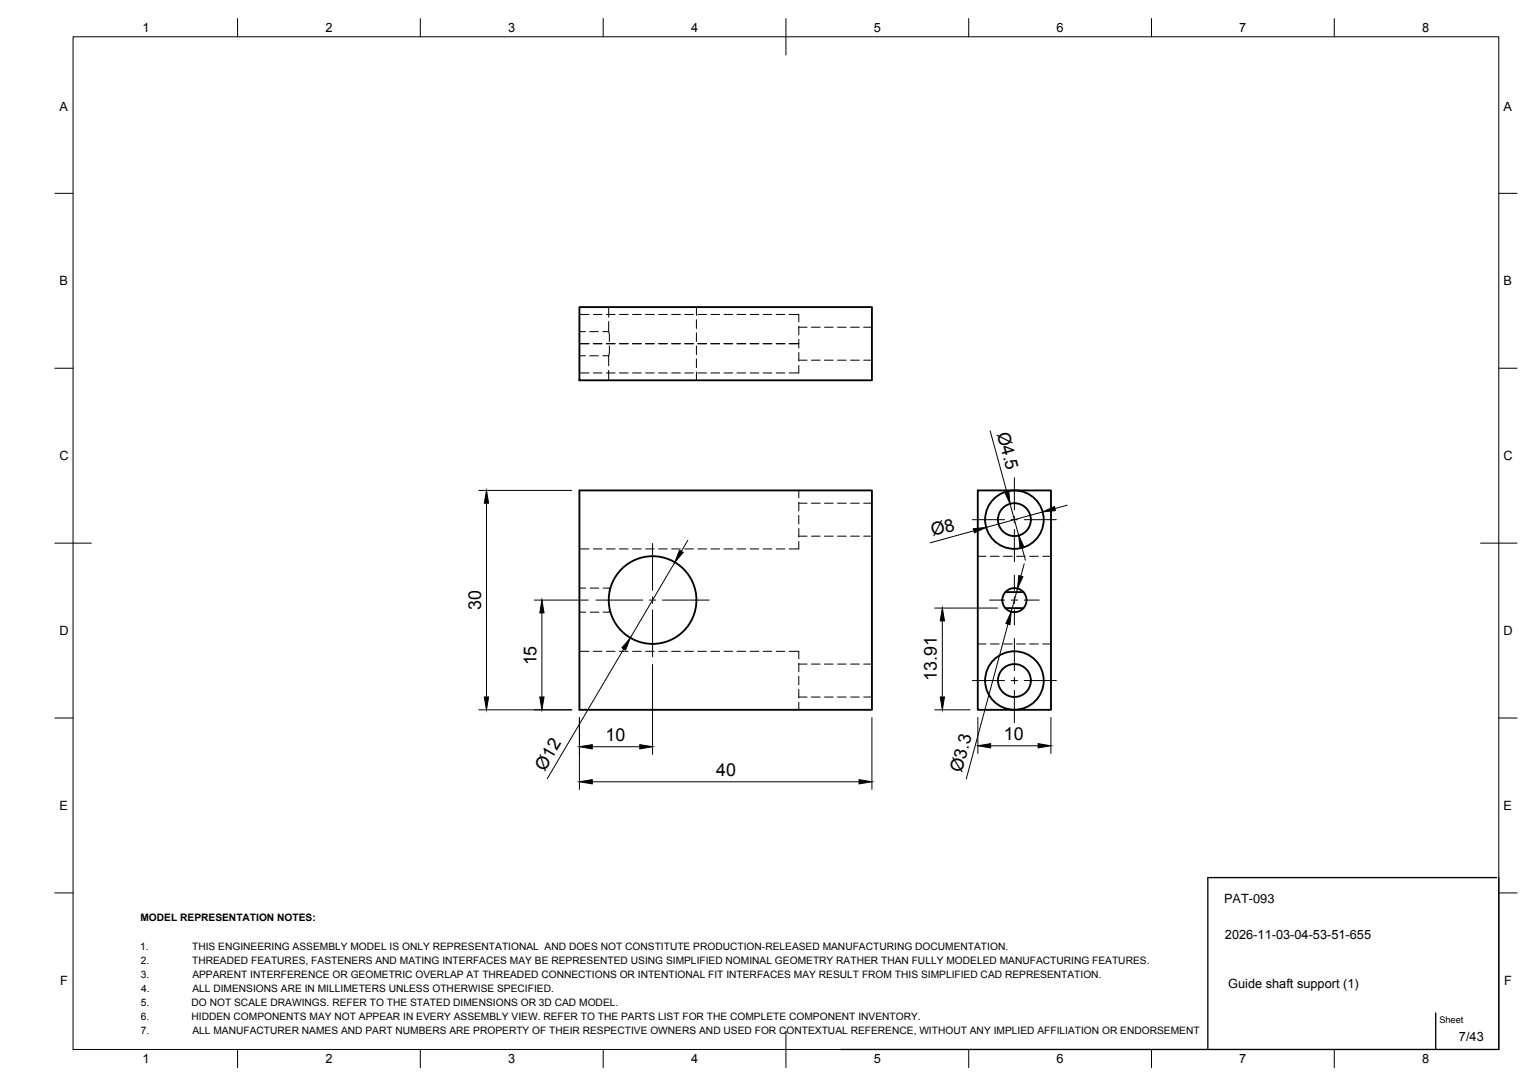
ISO-10303-21;
HEADER;
/* Generated by software containing ST-Developer
 * from STEP Tools, Inc. (www.steptools.com) 
 */

FILE_DESCRIPTION(
/* description */ ('Self-centering screw clamp'),
/* implementation_level */ '2;1');

FILE_NAME(
/* name */ 'Guide shaft support (1).step',
/* time_stamp */ '2026-10-28T03:25:31-07:00',
/* author */ (''),
/* organization */ (''),
/* preprocessor_version */ 'ST-DEVELOPER v20.2',
/* originating_system */ 'Autodesk Translation Framework v15.17.0.0',
/* authorisation */ '');

FILE_SCHEMA (('AUTOMOTIVE_DESIGN { 1 0 10303 214 3 1 1 }'));
ENDSEC;

DATA;
#10=MECHANICAL_DESIGN_GEOMETRIC_PRESENTATION_REPRESENTATION('',(#628),#16799);
#502=B_SPLINE_CURVE_WITH_KNOTS('',3,(#13973,#13974,#13975,#13976,#13977,
#13978),.UNSPECIFIED.,.F.,.F.,(4,2,4),(0.635430324955931,0.687528937234027,
0.750024497760672),.UNSPECIFIED.);
#503=B_SPLINE_CURVE_WITH_KNOTS('',3,(#13982,#13983,#13984,#13985,#13986,
#13987),.UNSPECIFIED.,.F.,.F.,(4,2,4),(0.250008165920224,0.312503726446869,
0.364602338724963),.UNSPECIFIED.);
#504=B_SPLINE_CURVE_WITH_KNOTS('',3,(#13988,#13989,#13990,#13991,#13992,
#13993),.UNSPECIFIED.,.F.,.F.,(4,2,4),(0.135413993115483,0.187512605393579,
0.250008165920224),.UNSPECIFIED.);
#505=B_SPLINE_CURVE_WITH_KNOTS('',3,(#13994,#13995,#13996,#13997,#13998,
#13999),.UNSPECIFIED.,.F.,.F.,(4,2,4),(0.750024497760672,0.812520058287317,
0.864618670565414),.UNSPECIFIED.);
#546=SHAPE_REPRESENTATION_RELATIONSHIP('SRR','None',#17019,#587);
#587=ADVANCED_BREP_SHAPE_REPRESENTATION('',(#676),#16757);
#628=STYLED_ITEM('',(#17326),#676);
#676=MANIFOLD_SOLID_BREP('Body1',#9079);
#749=FACE_BOUND('',#1863,.T.);
#750=FACE_BOUND('',#1866,.T.);
#751=FACE_BOUND('',#1868,.T.);
#752=FACE_BOUND('',#1874,.T.);
#753=FACE_BOUND('',#1877,.T.);
#754=FACE_BOUND('',#1879,.T.);
#755=FACE_BOUND('',#1880,.T.);
#1042=PLANE('',#9679);
#1043=PLANE('',#9684);
#1044=PLANE('',#9688);
#1045=PLANE('',#9693);
#1046=PLANE('',#9695);
#1047=PLANE('',#9703);
#1048=PLANE('',#9704);
#1049=PLANE('',#9705);
#1050=PLANE('',#9706);
#1051=PLANE('',#9707);
#1321=FACE_OUTER_BOUND('',#1856,.T.);
#1322=FACE_OUTER_BOUND('',#1857,.T.);
#1323=FACE_OUTER_BOUND('',#1858,.T.);
#1324=FACE_OUTER_BOUND('',#1859,.T.);
#1325=FACE_OUTER_BOUND('',#1860,.T.);
#1326=FACE_OUTER_BOUND('',#1861,.T.);
#1327=FACE_OUTER_BOUND('',#1862,.T.);
#1328=FACE_OUTER_BOUND('',#1864,.T.);
#1329=FACE_OUTER_BOUND('',#1865,.T.);
#1330=FACE_OUTER_BOUND('',#1867,.T.);
#1331=FACE_OUTER_BOUND('',#1869,.T.);
#1332=FACE_OUTER_BOUND('',#1870,.T.);
#1333=FACE_OUTER_BOUND('',#1871,.T.);
#1334=FACE_OUTER_BOUND('',#1872,.T.);
#1335=FACE_OUTER_BOUND('',#1873,.T.);
#1336=FACE_OUTER_BOUND('',#1875,.T.);
#1337=FACE_OUTER_BOUND('',#1876,.T.);
#1338=FACE_OUTER_BOUND('',#1878,.T.);
#1856=EDGE_LOOP('',(#6343,#6344,#6345,#6346));
#1857=EDGE_LOOP('',(#6347,#6348,#6349,#6350));
#1858=EDGE_LOOP('',(#6351,#6352));
#1859=EDGE_LOOP('',(#6353,#6354,#6355,#6356,#6357,#6358,#6359,#6360,#6361));
#1860=EDGE_LOOP('',(#6362,#6363));
#1861=EDGE_LOOP('',(#6364,#6365,#6366,#6367));
#1862=EDGE_LOOP('',(#6368,#6369));
#1863=EDGE_LOOP('',(#6370));
#1864=EDGE_LOOP('',(#6371,#6372,#6373,#6374));
#1865=EDGE_LOOP('',(#6375,#6376));
#1866=EDGE_LOOP('',(#6377));
#1867=EDGE_LOOP('',(#6378,#6379,#6380,#6381,#6382,#6383,#6384,#6385,#6386,
#6387));
#1868=EDGE_LOOP('',(#6388));
#1869=EDGE_LOOP('',(#6389,#6390,#6391,#6392));
#1870=EDGE_LOOP('',(#6393,#6394,#6395,#6396));
#1871=EDGE_LOOP('',(#6397,#6398,#6399,#6400,#6401,#6402,#6403,#6404,#6405,
#6406,#6407,#6408));
#1872=EDGE_LOOP('',(#6409,#6410,#6411,#6412,#6413,#6414,#6415));
#1873=EDGE_LOOP('',(#6416,#6417,#6418,#6419));
#1874=EDGE_LOOP('',(#6420));
#1875=EDGE_LOOP('',(#6421,#6422,#6423,#6424,#6425,#6426,#6427));
#1876=EDGE_LOOP('',(#6428,#6429,#6430,#6431));
#1877=EDGE_LOOP('',(#6432));
#1878=EDGE_LOOP('',(#6433,#6434,#6435,#6436));
#1879=EDGE_LOOP('',(#6437));
#1880=EDGE_LOOP('',(#6438));
#2652=LINE('',#13950,#3225);
#2653=LINE('',#13954,#3226);
#2654=LINE('',#13959,#3227);
#2655=LINE('',#13963,#3228);
#2656=LINE('',#13968,#3229);
#2657=LINE('',#14001,#3230);
#2658=LINE('',#14004,#3231);
#2659=LINE('',#14007,#3232);
#2660=LINE('',#14014,#3233);
#2661=LINE('',#14022,#3234);
#2662=LINE('',#14023,#3235);
#2663=LINE('',#14025,#3236);
#2664=LINE('',#14027,#3237);
#2665=LINE('',#14028,#3238);
#2666=LINE('',#14029,#3239);
#2667=LINE('',#14033,#3240);
#2668=LINE('',#14037,#3241);
#2669=LINE('',#14041,#3242);
#2670=LINE('',#14043,#3243);
#2671=LINE('',#14048,#3244);
#2672=LINE('',#14049,#3245);
#2673=LINE('',#14050,#3246);
#2674=LINE('',#14053,#3247);
#2675=LINE('',#14054,#3248);
#2676=LINE('',#14057,#3249);
#2677=LINE('',#14058,#3250);
#2678=LINE('',#14060,#3251);
#3225=VECTOR('',#11021,0.4);
#3226=VECTOR('',#11024,1.);
#3227=VECTOR('',#11029,0.4);
#3228=VECTOR('',#11032,1.);
#3229=VECTOR('',#11037,1.);
#3230=VECTOR('',#11044,0.164999999999999);
#3231=VECTOR('',#11049,1.);
#3232=VECTOR('',#11054,1.);
#3233=VECTOR('',#11065,1.);
#3234=VECTOR('',#11074,1.);
#3235=VECTOR('',#11075,1.);
#3236=VECTOR('',#11076,1.);
#3237=VECTOR('',#11077,1.);
#3238=VECTOR('',#11078,1.);
#3239=VECTOR('',#11079,1.);
#3240=VECTOR('',#11084,0.225);
#3241=VECTOR('',#11089,0.225);
#3242=VECTOR('',#11094,0.6);
#3243=VECTOR('',#11095,0.6);
#3244=VECTOR('',#11100,1.);
#3245=VECTOR('',#11101,1.);
#3246=VECTOR('',#11102,1.);
#3247=VECTOR('',#11105,1.);
#3248=VECTOR('',#11106,1.);
#3249=VECTOR('',#11109,1.);
#3250=VECTOR('',#11110,1.);
#3251=VECTOR('',#11113,1.);
#3764=CIRCLE('',#9674,0.4);
#3765=CIRCLE('',#9675,0.4);
#3766=CIRCLE('',#9677,0.4);
#3767=CIRCLE('',#9678,0.4);
#3768=CIRCLE('',#9680,0.164999999999999);
#3769=CIRCLE('',#9682,0.164999999999999);
#3770=CIRCLE('',#9683,0.164999999999999);
#3771=CIRCLE('',#9686,0.4);
#3772=CIRCLE('',#9687,0.4);
#3773=CIRCLE('',#9689,0.225);
#3774=CIRCLE('',#9691,0.4);
#3775=CIRCLE('',#9692,0.4);
#3776=CIRCLE('',#9694,0.225);
#3777=CIRCLE('',#9697,0.225);
#3778=CIRCLE('',#9699,0.225);
#3779=CIRCLE('',#9701,0.6);
#3780=CIRCLE('',#9702,0.6);
#4310=VERTEX_POINT('',#13948);
#4311=VERTEX_POINT('',#13949);
#4312=VERTEX_POINT('',#13951);
#4313=VERTEX_POINT('',#13953);
#4314=VERTEX_POINT('',#13957);
#4315=VERTEX_POINT('',#13958);
#4316=VERTEX_POINT('',#13960);
#4317=VERTEX_POINT('',#13962);
#4318=VERTEX_POINT('',#13966);
#4319=VERTEX_POINT('',#13967);
#4320=VERTEX_POINT('',#13971);
#4321=VERTEX_POINT('',#13972);
#4322=VERTEX_POINT('',#13979);
#4323=VERTEX_POINT('',#13981);
#4324=VERTEX_POINT('',#14000);
#4325=VERTEX_POINT('',#14010);
#4326=VERTEX_POINT('',#14017);
#4327=VERTEX_POINT('',#14020);
#4328=VERTEX_POINT('',#14021);
#4329=VERTEX_POINT('',#14024);
#4330=VERTEX_POINT('',#14026);
#4331=VERTEX_POINT('',#14031);
#4332=VERTEX_POINT('',#14035);
#4333=VERTEX_POINT('',#14039);
#4334=VERTEX_POINT('',#14042);
#4335=VERTEX_POINT('',#14046);
#4336=VERTEX_POINT('',#14047);
#4337=VERTEX_POINT('',#14052);
#4338=VERTEX_POINT('',#14056);
#5096=EDGE_CURVE('',#4310,#4311,#2652,.T.);
#5097=EDGE_CURVE('',#4312,#4310,#3764,.T.);
#5098=EDGE_CURVE('',#4312,#4313,#2653,.T.);
#5099=EDGE_CURVE('',#4311,#4313,#3765,.T.);
#5100=EDGE_CURVE('',#4314,#4315,#2654,.T.);
#5101=EDGE_CURVE('',#4316,#4314,#3766,.T.);
#5102=EDGE_CURVE('',#4316,#4317,#2655,.T.);
#5103=EDGE_CURVE('',#4315,#4317,#3767,.T.);
#5104=EDGE_CURVE('',#4318,#4319,#2656,.T.);
#5105=EDGE_CURVE('',#4318,#4319,#3768,.T.);
#5106=EDGE_CURVE('',#4320,#4321,#502,.T.);
#5107=EDGE_CURVE('',#4322,#4320,#3769,.T.);
#5108=EDGE_CURVE('',#4323,#4322,#503,.T.);
#5109=EDGE_CURVE('',#4319,#4323,#504,.T.);
#5110=EDGE_CURVE('',#4321,#4318,#505,.T.);
#5111=EDGE_CURVE('',#4321,#4324,#2657,.T.);
#5112=EDGE_CURVE('',#4324,#4324,#3770,.T.);
#5113=EDGE_CURVE('',#4322,#4320,#2658,.T.);
#5114=EDGE_CURVE('',#4317,#4315,#3771,.T.);
#5115=EDGE_CURVE('',#4316,#4317,#2659,.T.);
#5116=EDGE_CURVE('',#4314,#4316,#3772,.T.);
#5117=EDGE_CURVE('',#4325,#4325,#3773,.T.);
#5118=EDGE_CURVE('',#4313,#4311,#3774,.T.);
#5119=EDGE_CURVE('',#4312,#4313,#2660,.T.);
#5120=EDGE_CURVE('',#4310,#4312,#3775,.T.);
#5121=EDGE_CURVE('',#4326,#4326,#3776,.T.);
#5122=EDGE_CURVE('',#4327,#4328,#2661,.T.);
#5123=EDGE_CURVE('',#4328,#4317,#2662,.T.);
#5124=EDGE_CURVE('',#4317,#4329,#2663,.T.);
#5125=EDGE_CURVE('',#4329,#4330,#2664,.T.);
#5126=EDGE_CURVE('',#4330,#4313,#2665,.T.);
#5127=EDGE_CURVE('',#4313,#4327,#2666,.T.);
#5128=EDGE_CURVE('',#4331,#4331,#3777,.T.);
#5129=EDGE_CURVE('',#4331,#4325,#2667,.T.);
#5130=EDGE_CURVE('',#4332,#4332,#3778,.T.);
#5131=EDGE_CURVE('',#4332,#4326,#2668,.T.);
#5132=EDGE_CURVE('',#4333,#4333,#3779,.T.);
#5133=EDGE_CURVE('',#4333,#4321,#2669,.T.);
#5134=EDGE_CURVE('',#4323,#4334,#2670,.T.);
#5135=EDGE_CURVE('',#4334,#4334,#3780,.T.);
#5136=EDGE_CURVE('',#4335,#4336,#2671,.T.);
#5137=EDGE_CURVE('',#4336,#4327,#2672,.T.);
#5138=EDGE_CURVE('',#4335,#4330,#2673,.T.);
#5139=EDGE_CURVE('',#4337,#4335,#2674,.T.);
#5140=EDGE_CURVE('',#4337,#4329,#2675,.T.);
#5141=EDGE_CURVE('',#4338,#4337,#2676,.T.);
#5142=EDGE_CURVE('',#4338,#4328,#2677,.T.);
#5143=EDGE_CURVE('',#4336,#4338,#2678,.T.);
#6343=ORIENTED_EDGE('',*,*,#5096,.F.);
#6344=ORIENTED_EDGE('',*,*,#5097,.F.);
#6345=ORIENTED_EDGE('',*,*,#5098,.T.);
#6346=ORIENTED_EDGE('',*,*,#5099,.F.);
#6347=ORIENTED_EDGE('',*,*,#5100,.F.);
#6348=ORIENTED_EDGE('',*,*,#5101,.F.);
#6349=ORIENTED_EDGE('',*,*,#5102,.T.);
#6350=ORIENTED_EDGE('',*,*,#5103,.F.);
#6351=ORIENTED_EDGE('',*,*,#5104,.F.);
#6352=ORIENTED_EDGE('',*,*,#5105,.T.);
#6353=ORIENTED_EDGE('',*,*,#5106,.F.);
#6354=ORIENTED_EDGE('',*,*,#5107,.F.);
#6355=ORIENTED_EDGE('',*,*,#5108,.F.);
#6356=ORIENTED_EDGE('',*,*,#5109,.F.);
#6357=ORIENTED_EDGE('',*,*,#5105,.F.);
#6358=ORIENTED_EDGE('',*,*,#5110,.F.);
#6359=ORIENTED_EDGE('',*,*,#5111,.T.);
#6360=ORIENTED_EDGE('',*,*,#5112,.F.);
#6361=ORIENTED_EDGE('',*,*,#5111,.F.);
#6362=ORIENTED_EDGE('',*,*,#5113,.F.);
#6363=ORIENTED_EDGE('',*,*,#5107,.T.);
#6364=ORIENTED_EDGE('',*,*,#5100,.T.);
#6365=ORIENTED_EDGE('',*,*,#5114,.F.);
#6366=ORIENTED_EDGE('',*,*,#5115,.F.);
#6367=ORIENTED_EDGE('',*,*,#5116,.F.);
#6368=ORIENTED_EDGE('',*,*,#5101,.T.);
#6369=ORIENTED_EDGE('',*,*,#5116,.T.);
#6370=ORIENTED_EDGE('',*,*,#5117,.F.);
#6371=ORIENTED_EDGE('',*,*,#5096,.T.);
#6372=ORIENTED_EDGE('',*,*,#5118,.F.);
#6373=ORIENTED_EDGE('',*,*,#5119,.F.);
#6374=ORIENTED_EDGE('',*,*,#5120,.F.);
#6375=ORIENTED_EDGE('',*,*,#5097,.T.);
#6376=ORIENTED_EDGE('',*,*,#5120,.T.);
#6377=ORIENTED_EDGE('',*,*,#5121,.F.);
#6378=ORIENTED_EDGE('',*,*,#5122,.T.);
#6379=ORIENTED_EDGE('',*,*,#5123,.T.);
#6380=ORIENTED_EDGE('',*,*,#5114,.T.);
#6381=ORIENTED_EDGE('',*,*,#5103,.T.);
#6382=ORIENTED_EDGE('',*,*,#5124,.T.);
#6383=ORIENTED_EDGE('',*,*,#5125,.T.);
#6384=ORIENTED_EDGE('',*,*,#5126,.T.);
#6385=ORIENTED_EDGE('',*,*,#5118,.T.);
#6386=ORIENTED_EDGE('',*,*,#5099,.T.);
#6387=ORIENTED_EDGE('',*,*,#5127,.T.);
#6388=ORIENTED_EDGE('',*,*,#5112,.T.);
#6389=ORIENTED_EDGE('',*,*,#5128,.F.);
#6390=ORIENTED_EDGE('',*,*,#5129,.T.);
#6391=ORIENTED_EDGE('',*,*,#5117,.T.);
#6392=ORIENTED_EDGE('',*,*,#5129,.F.);
#6393=ORIENTED_EDGE('',*,*,#5130,.F.);
#6394=ORIENTED_EDGE('',*,*,#5131,.T.);
#6395=ORIENTED_EDGE('',*,*,#5121,.T.);
#6396=ORIENTED_EDGE('',*,*,#5131,.F.);
#6397=ORIENTED_EDGE('',*,*,#5132,.F.);
#6398=ORIENTED_EDGE('',*,*,#5133,.T.);
#6399=ORIENTED_EDGE('',*,*,#5110,.T.);
#6400=ORIENTED_EDGE('',*,*,#5104,.T.);
#6401=ORIENTED_EDGE('',*,*,#5109,.T.);
#6402=ORIENTED_EDGE('',*,*,#5134,.T.);
#6403=ORIENTED_EDGE('',*,*,#5135,.F.);
#6404=ORIENTED_EDGE('',*,*,#5134,.F.);
#6405=ORIENTED_EDGE('',*,*,#5108,.T.);
#6406=ORIENTED_EDGE('',*,*,#5113,.T.);
#6407=ORIENTED_EDGE('',*,*,#5106,.T.);
#6408=ORIENTED_EDGE('',*,*,#5133,.F.);
#6409=ORIENTED_EDGE('',*,*,#5136,.T.);
#6410=ORIENTED_EDGE('',*,*,#5137,.T.);
#6411=ORIENTED_EDGE('',*,*,#5127,.F.);
#6412=ORIENTED_EDGE('',*,*,#5098,.F.);
#6413=ORIENTED_EDGE('',*,*,#5119,.T.);
#6414=ORIENTED_EDGE('',*,*,#5126,.F.);
#6415=ORIENTED_EDGE('',*,*,#5138,.F.);
#6416=ORIENTED_EDGE('',*,*,#5139,.T.);
#6417=ORIENTED_EDGE('',*,*,#5138,.T.);
#6418=ORIENTED_EDGE('',*,*,#5125,.F.);
#6419=ORIENTED_EDGE('',*,*,#5140,.F.);
#6420=ORIENTED_EDGE('',*,*,#5135,.T.);
#6421=ORIENTED_EDGE('',*,*,#5141,.T.);
#6422=ORIENTED_EDGE('',*,*,#5140,.T.);
#6423=ORIENTED_EDGE('',*,*,#5124,.F.);
#6424=ORIENTED_EDGE('',*,*,#5102,.F.);
#6425=ORIENTED_EDGE('',*,*,#5115,.T.);
#6426=ORIENTED_EDGE('',*,*,#5123,.F.);
#6427=ORIENTED_EDGE('',*,*,#5142,.F.);
#6428=ORIENTED_EDGE('',*,*,#5143,.T.);
#6429=ORIENTED_EDGE('',*,*,#5142,.T.);
#6430=ORIENTED_EDGE('',*,*,#5122,.F.);
#6431=ORIENTED_EDGE('',*,*,#5137,.F.);
#6432=ORIENTED_EDGE('',*,*,#5132,.T.);
#6433=ORIENTED_EDGE('',*,*,#5143,.F.);
#6434=ORIENTED_EDGE('',*,*,#5136,.F.);
#6435=ORIENTED_EDGE('',*,*,#5139,.F.);
#6436=ORIENTED_EDGE('',*,*,#5141,.F.);
#6437=ORIENTED_EDGE('',*,*,#5128,.T.);
#6438=ORIENTED_EDGE('',*,*,#5130,.T.);
#8377=CYLINDRICAL_SURFACE('',#9673,0.4);
#8378=CYLINDRICAL_SURFACE('',#9676,0.4);
#8379=CYLINDRICAL_SURFACE('',#9681,0.164999999999999);
#8380=CYLINDRICAL_SURFACE('',#9685,0.4);
#8381=CYLINDRICAL_SURFACE('',#9690,0.4);
#8382=CYLINDRICAL_SURFACE('',#9696,0.225);
#8383=CYLINDRICAL_SURFACE('',#9698,0.225);
#8384=CYLINDRICAL_SURFACE('',#9700,0.6);
#8619=ADVANCED_FACE('',(#1321),#8377,.F.);
#8620=ADVANCED_FACE('',(#1322),#8378,.F.);
#8621=ADVANCED_FACE('',(#1323),#1042,.T.);
#8622=ADVANCED_FACE('',(#1324),#8379,.F.);
#8623=ADVANCED_FACE('',(#1325),#1043,.T.);
#8624=ADVANCED_FACE('',(#1326),#8380,.F.);
#8625=ADVANCED_FACE('',(#1327,#749),#1044,.T.);
#8626=ADVANCED_FACE('',(#1328),#8381,.F.);
#8627=ADVANCED_FACE('',(#1329,#750),#1045,.T.);
#8628=ADVANCED_FACE('',(#1330,#751),#1046,.T.);
#8629=ADVANCED_FACE('',(#1331),#8382,.F.);
#8630=ADVANCED_FACE('',(#1332),#8383,.F.);
#8631=ADVANCED_FACE('',(#1333),#8384,.F.);
#8632=ADVANCED_FACE('',(#1334),#1047,.T.);
#8633=ADVANCED_FACE('',(#1335,#752),#1048,.T.);
#8634=ADVANCED_FACE('',(#1336),#1049,.T.);
#8635=ADVANCED_FACE('',(#1337,#753),#1050,.T.);
#8636=ADVANCED_FACE('',(#1338,#754,#755),#1051,.F.);
#9079=CLOSED_SHELL('',(#8619,#8620,#8621,#8622,#8623,#8624,#8625,#8626,
#8627,#8628,#8629,#8630,#8631,#8632,#8633,#8634,#8635,#8636));
#9672=AXIS2_PLACEMENT_3D('',#13946,#11017,#11018);
#9673=AXIS2_PLACEMENT_3D('',#13947,#11019,#11020);
#9674=AXIS2_PLACEMENT_3D('',#13952,#11022,#11023);
#9675=AXIS2_PLACEMENT_3D('',#13955,#11025,#11026);
#9676=AXIS2_PLACEMENT_3D('',#13956,#11027,#11028);
#9677=AXIS2_PLACEMENT_3D('',#13961,#11030,#11031);
#9678=AXIS2_PLACEMENT_3D('',#13964,#11033,#11034);
#9679=AXIS2_PLACEMENT_3D('',#13965,#11035,#11036);
#9680=AXIS2_PLACEMENT_3D('',#13969,#11038,#11039);
#9681=AXIS2_PLACEMENT_3D('',#13970,#11040,#11041);
#9682=AXIS2_PLACEMENT_3D('',#13980,#11042,#11043);
#9683=AXIS2_PLACEMENT_3D('',#14002,#11045,#11046);
#9684=AXIS2_PLACEMENT_3D('',#14003,#11047,#11048);
#9685=AXIS2_PLACEMENT_3D('',#14005,#11050,#11051);
#9686=AXIS2_PLACEMENT_3D('',#14006,#11052,#11053);
#9687=AXIS2_PLACEMENT_3D('',#14008,#11055,#11056);
#9688=AXIS2_PLACEMENT_3D('',#14009,#11057,#11058);
#9689=AXIS2_PLACEMENT_3D('',#14011,#11059,#11060);
#9690=AXIS2_PLACEMENT_3D('',#14012,#11061,#11062);
#9691=AXIS2_PLACEMENT_3D('',#14013,#11063,#11064);
#9692=AXIS2_PLACEMENT_3D('',#14015,#11066,#11067);
#9693=AXIS2_PLACEMENT_3D('',#14016,#11068,#11069);
#9694=AXIS2_PLACEMENT_3D('',#14018,#11070,#11071);
#9695=AXIS2_PLACEMENT_3D('',#14019,#11072,#11073);
#9696=AXIS2_PLACEMENT_3D('',#14030,#11080,#11081);
#9697=AXIS2_PLACEMENT_3D('',#14032,#11082,#11083);
#9698=AXIS2_PLACEMENT_3D('',#14034,#11085,#11086);
#9699=AXIS2_PLACEMENT_3D('',#14036,#11087,#11088);
#9700=AXIS2_PLACEMENT_3D('',#14038,#11090,#11091);
#9701=AXIS2_PLACEMENT_3D('',#14040,#11092,#11093);
#9702=AXIS2_PLACEMENT_3D('',#14044,#11096,#11097);
#9703=AXIS2_PLACEMENT_3D('',#14045,#11098,#11099);
#9704=AXIS2_PLACEMENT_3D('',#14051,#11103,#11104);
#9705=AXIS2_PLACEMENT_3D('',#14055,#11107,#11108);
#9706=AXIS2_PLACEMENT_3D('',#14059,#11111,#11112);
#9707=AXIS2_PLACEMENT_3D('',#14061,#11114,#11115);
#11017=DIRECTION('axis',(0.,0.,1.));
#11018=DIRECTION('refdir',(1.,0.,0.));
#11019=DIRECTION('center_axis',(0.,0.,1.));
#11020=DIRECTION('ref_axis',(1.,0.,0.));
#11021=DIRECTION('',(0.,0.,1.));
#11022=DIRECTION('center_axis',(0.,0.,1.));
#11023=DIRECTION('ref_axis',(1.,0.,0.));
#11024=DIRECTION('',(0.,0.,1.));
#11025=DIRECTION('center_axis',(0.,0.,-1.));
#11026=DIRECTION('ref_axis',(1.,0.,0.));
#11027=DIRECTION('center_axis',(0.,0.,1.));
#11028=DIRECTION('ref_axis',(1.,0.,0.));
#11029=DIRECTION('',(0.,0.,1.));
#11030=DIRECTION('center_axis',(0.,0.,1.));
#11031=DIRECTION('ref_axis',(1.,0.,0.));
#11032=DIRECTION('',(0.,0.,1.));
#11033=DIRECTION('center_axis',(0.,0.,-1.));
#11034=DIRECTION('ref_axis',(1.,0.,0.));
#11035=DIRECTION('center_axis',(0.,0.,1.));
#11036=DIRECTION('ref_axis',(1.,0.,0.));
#11037=DIRECTION('',(1.,0.,0.));
#11038=DIRECTION('center_axis',(0.,0.,1.));
#11039=DIRECTION('ref_axis',(1.,0.,0.));
#11040=DIRECTION('center_axis',(0.,0.,1.));
#11041=DIRECTION('ref_axis',(1.,0.,0.));
#11042=DIRECTION('center_axis',(0.,0.,1.));
#11043=DIRECTION('ref_axis',(1.,0.,0.));
#11044=DIRECTION('',(0.,0.,1.));
#11045=DIRECTION('center_axis',(0.,0.,-1.));
#11046=DIRECTION('ref_axis',(1.,0.,0.));
#11047=DIRECTION('center_axis',(0.,0.,1.));
#11048=DIRECTION('ref_axis',(1.,0.,0.));
#11049=DIRECTION('',(-1.,0.,0.));
#11050=DIRECTION('center_axis',(0.,0.,1.));
#11051=DIRECTION('ref_axis',(1.,0.,0.));
#11052=DIRECTION('center_axis',(0.,0.,-1.));
#11053=DIRECTION('ref_axis',(1.,0.,0.));
#11054=DIRECTION('',(0.,0.,1.));
#11055=DIRECTION('center_axis',(0.,0.,1.));
#11056=DIRECTION('ref_axis',(1.,0.,0.));
#11057=DIRECTION('center_axis',(0.,0.,1.));
#11058=DIRECTION('ref_axis',(1.,0.,0.));
#11059=DIRECTION('center_axis',(0.,0.,1.));
#11060=DIRECTION('ref_axis',(1.,0.,0.));
#11061=DIRECTION('center_axis',(0.,0.,1.));
#11062=DIRECTION('ref_axis',(1.,0.,0.));
#11063=DIRECTION('center_axis',(0.,0.,-1.));
#11064=DIRECTION('ref_axis',(1.,0.,0.));
#11065=DIRECTION('',(0.,0.,1.));
#11066=DIRECTION('center_axis',(0.,0.,1.));
#11067=DIRECTION('ref_axis',(1.,0.,0.));
#11068=DIRECTION('center_axis',(0.,0.,1.));
#11069=DIRECTION('ref_axis',(1.,0.,0.));
#11070=DIRECTION('center_axis',(0.,0.,1.));
#11071=DIRECTION('ref_axis',(1.,0.,0.));
#11072=DIRECTION('center_axis',(0.,0.,1.));
#11073=DIRECTION('ref_axis',(1.,0.,0.));
#11074=DIRECTION('',(0.,-1.,0.));
#11075=DIRECTION('',(1.,0.,0.));
#11076=DIRECTION('',(1.,0.,0.));
#11077=DIRECTION('',(0.,1.,0.));
#11078=DIRECTION('',(-1.,0.,0.));
#11079=DIRECTION('',(-1.,0.,0.));
#11080=DIRECTION('center_axis',(0.,0.,1.));
#11081=DIRECTION('ref_axis',(1.,0.,0.));
#11082=DIRECTION('center_axis',(0.,0.,1.));
#11083=DIRECTION('ref_axis',(1.,0.,0.));
#11084=DIRECTION('',(0.,0.,1.));
#11085=DIRECTION('center_axis',(0.,0.,1.));
#11086=DIRECTION('ref_axis',(1.,0.,0.));
#11087=DIRECTION('center_axis',(0.,0.,1.));
#11088=DIRECTION('ref_axis',(1.,0.,0.));
#11089=DIRECTION('',(0.,0.,1.));
#11090=DIRECTION('center_axis',(1.,0.,0.));
#11091=DIRECTION('ref_axis',(0.,0.,-1.));
#11092=DIRECTION('center_axis',(1.,0.,0.));
#11093=DIRECTION('ref_axis',(0.,0.,-1.));
#11094=DIRECTION('',(1.,0.,0.));
#11095=DIRECTION('',(1.,0.,0.));
#11096=DIRECTION('center_axis',(-1.,0.,0.));
#11097=DIRECTION('ref_axis',(0.,0.,-1.));
#11098=DIRECTION('center_axis',(0.,1.,0.));
#11099=DIRECTION('ref_axis',(-1.,0.,0.));
#11100=DIRECTION('',(-1.,0.,0.));
#11101=DIRECTION('',(0.,0.,1.));
#11102=DIRECTION('',(0.,0.,1.));
#11103=DIRECTION('center_axis',(1.,0.,0.));
#11104=DIRECTION('ref_axis',(0.,1.,0.));
#11105=DIRECTION('',(0.,1.,0.));
#11106=DIRECTION('',(0.,0.,1.));
#11107=DIRECTION('center_axis',(0.,-1.,0.));
#11108=DIRECTION('ref_axis',(1.,0.,0.));
#11109=DIRECTION('',(1.,0.,0.));
#11110=DIRECTION('',(0.,0.,1.));
#11111=DIRECTION('center_axis',(-1.,0.,0.));
#11112=DIRECTION('ref_axis',(0.,-1.,0.));
#11113=DIRECTION('',(0.,-1.,0.));
#11114=DIRECTION('center_axis',(0.,0.,1.));
#11115=DIRECTION('ref_axis',(1.,0.,0.));
#13946=CARTESIAN_POINT('',(0.,0.,0.));
#13947=CARTESIAN_POINT('Origin',(13.5,-1.9,2.));
#13948=CARTESIAN_POINT('',(13.1,-1.9,2.));
#13949=CARTESIAN_POINT('',(13.1,-1.9,5.));
#13950=CARTESIAN_POINT('',(13.1,-1.9,2.));
#13951=CARTESIAN_POINT('',(13.5,-1.5,2.));
#13952=CARTESIAN_POINT('Origin',(13.5,-1.9,2.));
#13953=CARTESIAN_POINT('',(13.5,-1.5,5.));
#13954=CARTESIAN_POINT('',(13.5,-1.5,2.));
#13955=CARTESIAN_POINT('Origin',(13.5,-1.9,5.));
#13956=CARTESIAN_POINT('Origin',(13.5,-4.1,2.));
#13957=CARTESIAN_POINT('',(13.1,-4.1,2.));
#13958=CARTESIAN_POINT('',(13.1,-4.1,5.));
#13959=CARTESIAN_POINT('',(13.1,-4.1,2.));
#13960=CARTESIAN_POINT('',(13.5,-4.5,2.));
#13961=CARTESIAN_POINT('Origin',(13.5,-4.1,2.));
#13962=CARTESIAN_POINT('',(13.5,-4.5,5.));
#13963=CARTESIAN_POINT('',(13.5,-4.5,2.));
#13964=CARTESIAN_POINT('Origin',(13.5,-4.1,5.));
#13965=CARTESIAN_POINT('Origin',(13.5,-3.,4.59));
#13966=CARTESIAN_POINT('',(13.3762058159686,-3.10908712114636,4.59));
#13967=CARTESIAN_POINT('',(13.6237941840314,-3.10908712114636,4.59));
#13968=CARTESIAN_POINT('',(12.9,-3.10908712114636,4.59));
#13969=CARTESIAN_POINT('Origin',(13.5,-3.,4.59));
#13970=CARTESIAN_POINT('Origin',(13.5,-3.,4.59));
#13971=CARTESIAN_POINT('',(13.3762058159686,-2.89091287885364,4.59));
#13972=CARTESIAN_POINT('',(13.335,-3.,4.6));
#13973=CARTESIAN_POINT('Ctrl Pts',(13.3762058159686,-2.89091287885364,4.59));
#13974=CARTESIAN_POINT('Ctrl Pts',(13.3646008648105,-2.90408240284739,4.59243495840567));
#13975=CARTESIAN_POINT('Ctrl Pts',(13.3546543563418,-2.91977655056228,4.59485638705045));
#13976=CARTESIAN_POINT('Ctrl Pts',(13.339185135366,-2.95701983403981,4.59880705606552));
#13977=CARTESIAN_POINT('Ctrl Pts',(13.335,-2.97916814649112,4.6));
#13978=CARTESIAN_POINT('Ctrl Pts',(13.335,-3.,4.6));
#13979=CARTESIAN_POINT('',(13.6237941840314,-2.89091287885364,4.59));
#13980=CARTESIAN_POINT('Origin',(13.5,-3.,4.59));
#13981=CARTESIAN_POINT('',(13.665,-3.,4.6));
#13982=CARTESIAN_POINT('Ctrl Pts',(13.665,-3.,4.6));
#13983=CARTESIAN_POINT('Ctrl Pts',(13.665,-2.97916814649112,4.6));
#13984=CARTESIAN_POINT('Ctrl Pts',(13.660814864634,-2.95701983403981,4.59880705606552));
#13985=CARTESIAN_POINT('Ctrl Pts',(13.6453456436582,-2.91977655056228,4.59485638705045));
#13986=CARTESIAN_POINT('Ctrl Pts',(13.6353991351895,-2.90408240284739,4.59243495840567));
#13987=CARTESIAN_POINT('Ctrl Pts',(13.6237941840314,-2.89091287885364,4.59));
#13988=CARTESIAN_POINT('Ctrl Pts',(13.6237941840314,-3.10908712114636,4.59));
#13989=CARTESIAN_POINT('Ctrl Pts',(13.6353991351895,-3.09591759715261,4.59243495840567));
#13990=CARTESIAN_POINT('Ctrl Pts',(13.6453456436582,-3.08022344943772,4.59485638705045));
#13991=CARTESIAN_POINT('Ctrl Pts',(13.660814864634,-3.04298016596019,4.59880705606552));
#13992=CARTESIAN_POINT('Ctrl Pts',(13.665,-3.02083185350888,4.6));
#13993=CARTESIAN_POINT('Ctrl Pts',(13.665,-3.,4.6));
#13994=CARTESIAN_POINT('Ctrl Pts',(13.335,-3.,4.6));
#13995=CARTESIAN_POINT('Ctrl Pts',(13.335,-3.02083185350888,4.6));
#13996=CARTESIAN_POINT('Ctrl Pts',(13.339185135366,-3.04298016596019,4.59880705606552));
#13997=CARTESIAN_POINT('Ctrl Pts',(13.3546543563418,-3.08022344943772,4.59485638705045));
#13998=CARTESIAN_POINT('Ctrl Pts',(13.3646008648105,-3.09591759715261,4.59243495840567));
#13999=CARTESIAN_POINT('Ctrl Pts',(13.3762058159686,-3.10908712114636,4.59));
#14000=CARTESIAN_POINT('',(13.335,-3.,5.));
#14001=CARTESIAN_POINT('',(13.335,-3.,4.59));
#14002=CARTESIAN_POINT('Origin',(13.5,-3.,5.));
#14003=CARTESIAN_POINT('Origin',(13.5,-3.,4.59));
#14004=CARTESIAN_POINT('',(12.9,-2.89091287885364,4.59));
#14005=CARTESIAN_POINT('Origin',(13.5,-4.1,2.));
#14006=CARTESIAN_POINT('Origin',(13.5,-4.1,5.));
#14007=CARTESIAN_POINT('',(13.5,-4.5,2.));
#14008=CARTESIAN_POINT('Origin',(13.5,-4.1,2.));
#14009=CARTESIAN_POINT('Origin',(13.5,-4.1,2.));
#14010=CARTESIAN_POINT('',(13.275,-4.1,2.));
#14011=CARTESIAN_POINT('Origin',(13.5,-4.1,2.));
#14012=CARTESIAN_POINT('Origin',(13.5,-1.9,2.));
#14013=CARTESIAN_POINT('Origin',(13.5,-1.9,5.));
#14014=CARTESIAN_POINT('',(13.5,-1.5,2.));
#14015=CARTESIAN_POINT('Origin',(13.5,-1.9,2.));
#14016=CARTESIAN_POINT('Origin',(13.5,-1.9,2.));
#14017=CARTESIAN_POINT('',(13.275,-1.9,2.));
#14018=CARTESIAN_POINT('Origin',(13.5,-1.9,2.));
#14019=CARTESIAN_POINT('Origin',(13.5,-3.,5.));
#14020=CARTESIAN_POINT('',(13.,-1.5,5.));
#14021=CARTESIAN_POINT('',(13.,-4.5,5.));
#14022=CARTESIAN_POINT('',(13.,-1.5,5.));
#14023=CARTESIAN_POINT('',(13.,-4.5,5.));
#14024=CARTESIAN_POINT('',(14.,-4.5,5.));
#14025=CARTESIAN_POINT('',(13.,-4.5,5.));
#14026=CARTESIAN_POINT('',(14.,-1.5,5.));
#14027=CARTESIAN_POINT('',(14.,-4.5,5.));
#14028=CARTESIAN_POINT('',(14.,-1.5,5.));
#14029=CARTESIAN_POINT('',(14.,-1.5,5.));
#14030=CARTESIAN_POINT('Origin',(13.5,-4.1,0.9));
#14031=CARTESIAN_POINT('',(13.275,-4.1,1.));
#14032=CARTESIAN_POINT('Origin',(13.5,-4.1,1.));
#14033=CARTESIAN_POINT('',(13.275,-4.1,0.9));
#14034=CARTESIAN_POINT('Origin',(13.5,-1.9,0.9));
#14035=CARTESIAN_POINT('',(13.275,-1.9,1.));
#14036=CARTESIAN_POINT('Origin',(13.5,-1.9,1.));
#14037=CARTESIAN_POINT('',(13.275,-1.9,0.9));
#14038=CARTESIAN_POINT('Origin',(12.9,-3.,4.));
#14039=CARTESIAN_POINT('',(13.,-3.,4.6));
#14040=CARTESIAN_POINT('Origin',(13.,-3.,4.));
#14041=CARTESIAN_POINT('',(12.9,-3.,4.6));
#14042=CARTESIAN_POINT('',(14.,-3.,4.6));
#14043=CARTESIAN_POINT('',(12.9,-3.,4.6));
#14044=CARTESIAN_POINT('Origin',(14.,-3.,4.));
#14045=CARTESIAN_POINT('Origin',(14.,-1.5,1.));
#14046=CARTESIAN_POINT('',(14.,-1.5,1.));
#14047=CARTESIAN_POINT('',(13.,-1.5,1.));
#14048=CARTESIAN_POINT('',(14.,-1.5,1.));
#14049=CARTESIAN_POINT('',(13.,-1.5,1.));
#14050=CARTESIAN_POINT('',(14.,-1.5,1.));
#14051=CARTESIAN_POINT('Origin',(14.,-4.5,1.));
#14052=CARTESIAN_POINT('',(14.,-4.5,1.));
#14053=CARTESIAN_POINT('',(14.,-4.5,1.));
#14054=CARTESIAN_POINT('',(14.,-4.5,1.));
#14055=CARTESIAN_POINT('Origin',(13.,-4.5,1.));
#14056=CARTESIAN_POINT('',(13.,-4.5,1.));
#14057=CARTESIAN_POINT('',(13.,-4.5,1.));
#14058=CARTESIAN_POINT('',(13.,-4.5,1.));
#14059=CARTESIAN_POINT('Origin',(13.,-1.5,1.));
#14060=CARTESIAN_POINT('',(13.,-1.5,1.));
#14061=CARTESIAN_POINT('Origin',(13.5,-3.,1.));
#16708=UNCERTAINTY_MEASURE_WITH_UNIT(LENGTH_MEASURE(0.001),#16800,
'DISTANCE_ACCURACY_VALUE',
'Maximum model space distance between geometric entities at asserted c
onnectivities');
#16750=UNCERTAINTY_MEASURE_WITH_UNIT(LENGTH_MEASURE(0.001),#16800,
'DISTANCE_ACCURACY_VALUE',
'Maximum model space distance between geometric entities at asserted c
onnectivities');
#16757=(
GEOMETRIC_REPRESENTATION_CONTEXT(3)
GLOBAL_UNCERTAINTY_ASSIGNED_CONTEXT((#16708))
GLOBAL_UNIT_ASSIGNED_CONTEXT((#16800,#16802,#16803))
REPRESENTATION_CONTEXT('','3D')
);
#16799=(
GEOMETRIC_REPRESENTATION_CONTEXT(3)
GLOBAL_UNCERTAINTY_ASSIGNED_CONTEXT((#16750))
GLOBAL_UNIT_ASSIGNED_CONTEXT((#16800,#16802,#16803))
REPRESENTATION_CONTEXT('','3D')
);
#16800=(
LENGTH_UNIT()
NAMED_UNIT(*)
SI_UNIT(.CENTI.,.METRE.)
);
#16802=(
NAMED_UNIT(*)
PLANE_ANGLE_UNIT()
SI_UNIT($,.RADIAN.)
);
#16803=(
NAMED_UNIT(*)
SI_UNIT($,.STERADIAN.)
SOLID_ANGLE_UNIT()
);
#16810=SHAPE_DEFINITION_REPRESENTATION(#16858,#17019);
#16858=PRODUCT_DEFINITION_SHAPE('',$,#17068);
#17019=SHAPE_REPRESENTATION('',(#9672),#16757);
#17061=PRODUCT_DEFINITION_CONTEXT('part definition',#17207,'design');
#17068=PRODUCT_DEFINITION('Guide shaft support (1)',
'Guide shaft support (1)',#17116,#17061);
#17116=PRODUCT_DEFINITION_FORMATION('',$,#17215);
#17207=APPLICATION_CONTEXT(
'Core Data for Automotive Mechanical Design Process');
#17208=PRODUCT_CONTEXT('part definition',#17207,'mechanical');
#17215=PRODUCT('Guide shaft support (1)','Guide shaft support (1)',
'Guide shaft support (1)',(#17208));
#17320=COLOUR_RGB('Grey',0.48,0.52,0.57);
#17321=FILL_AREA_STYLE_COLOUR('',#17320);
#17322=FILL_AREA_STYLE('',(#17321));
#17323=SURFACE_STYLE_FILL_AREA(#17322);
#17324=SURFACE_SIDE_STYLE('',(#17323));
#17325=SURFACE_STYLE_USAGE(.BOTH.,#17324);
#17326=PRESENTATION_STYLE_ASSIGNMENT((#17325));
ENDSEC;
END-ISO-10303-21;
